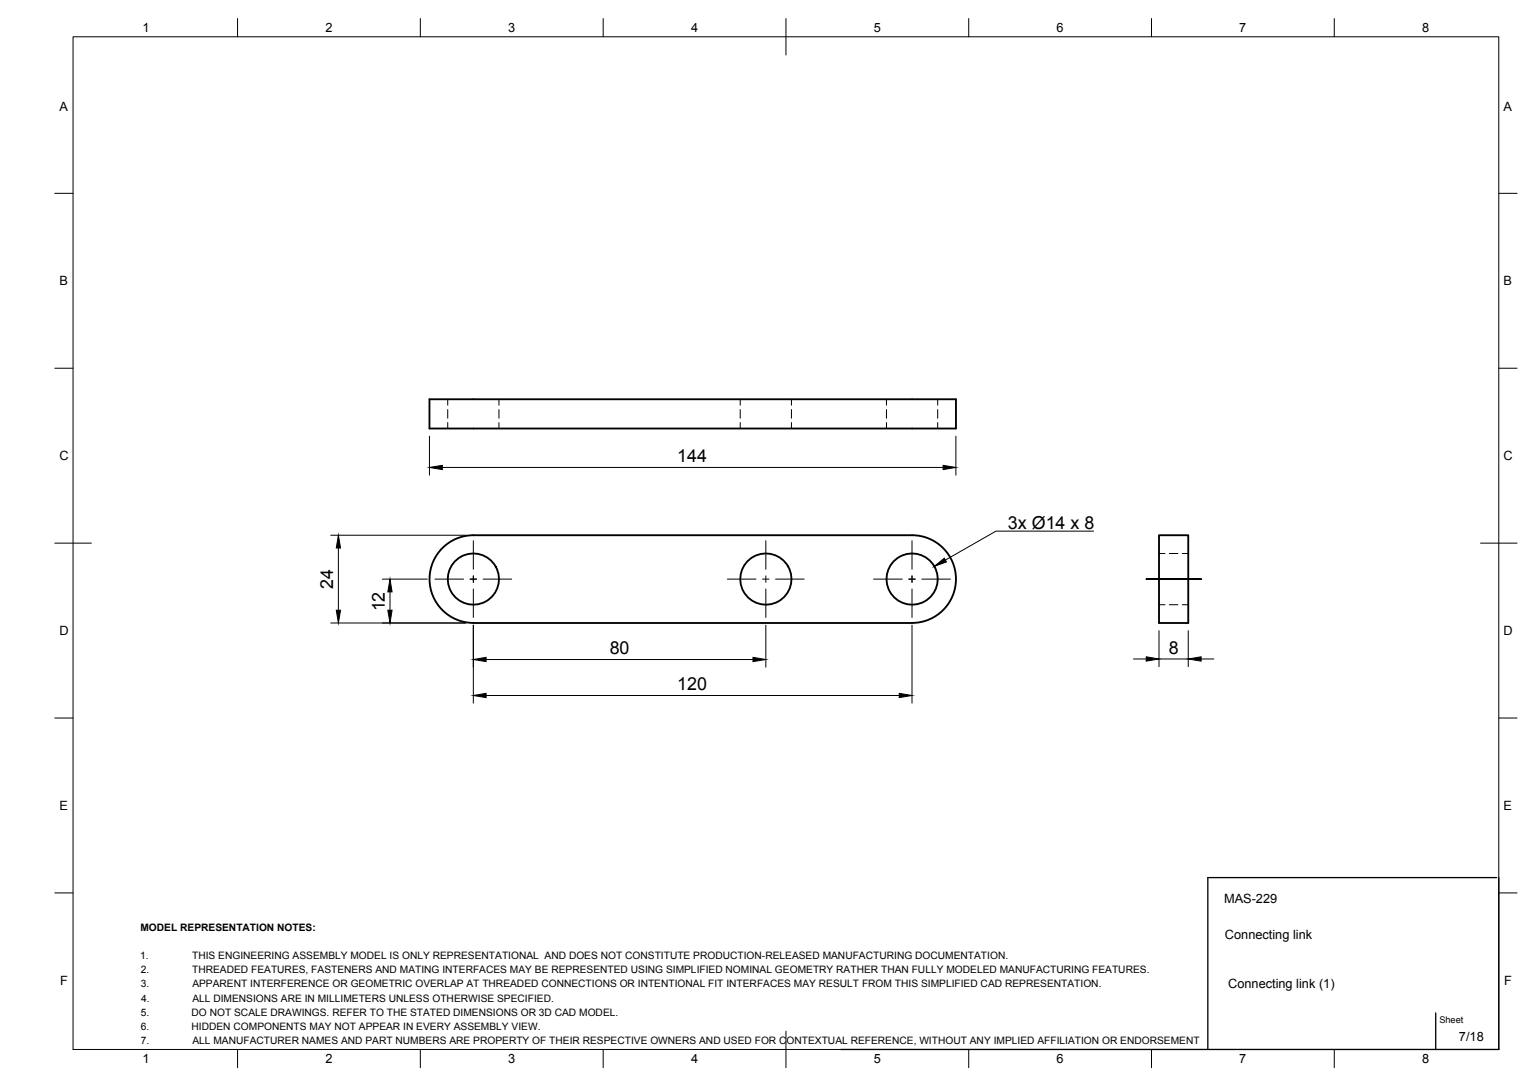
ISO-10303-21;
HEADER;
/* Generated by software containing ST-Developer
 * from STEP Tools, Inc. (www.steptools.com) 
 */

FILE_DESCRIPTION(
/* description */ ('Independently dimensioned six-bar single-leg walking-linkage demonstr
ator. Whole-mm20 crank,60 upper rocker,80/120 ternary coupler,120 lowe
r rocker,140 knee pitch and260 toe reach; ground pivots0/0,60/0,40/60.
 Seven native revolutes close both loops. Four reused native library f
amilies, fully retained shared pins and layered real spacer stacks, bo
nded rubber toe. Benchtop reference mechanism; no complete vehicle, lo
ad, gait stability, adhesive, weld, fit or life rating.'),
/* implementation_level */ '2;1');

FILE_NAME(
/* name */ 'Connecting link.step',
/* time_stamp */ '2026-11-09T20:33:14-08:00',
/* author */ (''),
/* organization */ (''),
/* preprocessor_version */ 'ST-DEVELOPER v20.2',
/* originating_system */ 'Autodesk Translation Framework v15.17.0.0',
/* authorisation */ '');

FILE_SCHEMA (('AUTOMOTIVE_DESIGN { 1 0 10303 214 3 1 1 }'));
ENDSEC;

DATA;
#10=MECHANICAL_DESIGN_GEOMETRIC_PRESENTATION_REPRESENTATION('',(#259),#4048);
#223=SHAPE_REPRESENTATION_RELATIONSHIP('SRR','None',#4147,#241);
#241=ADVANCED_BREP_SHAPE_REPRESENTATION('',(#277),#4034);
#259=STYLED_ITEM('',(#4246),#277);
#277=MANIFOLD_SOLID_BREP('Body1',#2148);
#313=FACE_BOUND('',#608,.T.);
#314=FACE_BOUND('',#609,.T.);
#315=FACE_BOUND('',#610,.T.);
#316=FACE_BOUND('',#612,.T.);
#317=FACE_BOUND('',#613,.T.);
#318=FACE_BOUND('',#614,.T.);
#370=PLANE('',#2443);
#371=PLANE('',#2447);
#372=PLANE('',#2451);
#373=PLANE('',#2452);
#452=FACE_OUTER_BOUND('',#600,.T.);
#453=FACE_OUTER_BOUND('',#601,.T.);
#454=FACE_OUTER_BOUND('',#602,.T.);
#455=FACE_OUTER_BOUND('',#603,.T.);
#456=FACE_OUTER_BOUND('',#604,.T.);
#457=FACE_OUTER_BOUND('',#605,.T.);
#458=FACE_OUTER_BOUND('',#606,.T.);
#459=FACE_OUTER_BOUND('',#607,.T.);
#460=FACE_OUTER_BOUND('',#611,.T.);
#600=EDGE_LOOP('',(#1659,#1660,#1661,#1662));
#601=EDGE_LOOP('',(#1663,#1664,#1665,#1666));
#602=EDGE_LOOP('',(#1667,#1668,#1669,#1670));
#603=EDGE_LOOP('',(#1671,#1672,#1673,#1674));
#604=EDGE_LOOP('',(#1675,#1676,#1677,#1678));
#605=EDGE_LOOP('',(#1679,#1680,#1681,#1682));
#606=EDGE_LOOP('',(#1683,#1684,#1685,#1686));
#607=EDGE_LOOP('',(#1687,#1688,#1689,#1690));
#608=EDGE_LOOP('',(#1691));
#609=EDGE_LOOP('',(#1692));
#610=EDGE_LOOP('',(#1693));
#611=EDGE_LOOP('',(#1694,#1695,#1696,#1697));
#612=EDGE_LOOP('',(#1698));
#613=EDGE_LOOP('',(#1699));
#614=EDGE_LOOP('',(#1700));
#781=LINE('',#3608,#906);
#782=LINE('',#3614,#907);
#783=LINE('',#3620,#908);
#784=LINE('',#3625,#909);
#785=LINE('',#3627,#910);
#786=LINE('',#3629,#911);
#787=LINE('',#3630,#912);
#788=LINE('',#3636,#913);
#789=LINE('',#3639,#914);
#790=LINE('',#3641,#915);
#791=LINE('',#3642,#916);
#906=VECTOR('',#2878,7.);
#907=VECTOR('',#2885,7.);
#908=VECTOR('',#2892,7.);
#909=VECTOR('',#2897,10.);
#910=VECTOR('',#2898,10.);
#911=VECTOR('',#2899,10.);
#912=VECTOR('',#2900,10.);
#913=VECTOR('',#2907,10.);
#914=VECTOR('',#2910,10.);
#915=VECTOR('',#2911,10.);
#916=VECTOR('',#2912,10.);
#1004=CIRCLE('',#2435,7.);
#1005=CIRCLE('',#2436,7.);
#1006=CIRCLE('',#2438,7.);
#1007=CIRCLE('',#2439,7.);
#1008=CIRCLE('',#2441,7.);
#1009=CIRCLE('',#2442,7.);
#1010=CIRCLE('',#2445,12.);
#1011=CIRCLE('',#2446,12.);
#1012=CIRCLE('',#2449,12.);
#1013=CIRCLE('',#2450,12.);
#1146=VERTEX_POINT('',#3605);
#1147=VERTEX_POINT('',#3607);
#1148=VERTEX_POINT('',#3611);
#1149=VERTEX_POINT('',#3613);
#1150=VERTEX_POINT('',#3617);
#1151=VERTEX_POINT('',#3619);
#1152=VERTEX_POINT('',#3623);
#1153=VERTEX_POINT('',#3624);
#1154=VERTEX_POINT('',#3626);
#1155=VERTEX_POINT('',#3628);
#1156=VERTEX_POINT('',#3632);
#1157=VERTEX_POINT('',#3634);
#1158=VERTEX_POINT('',#3638);
#1159=VERTEX_POINT('',#3640);
#1333=EDGE_CURVE('',#1146,#1146,#1004,.T.);
#1334=EDGE_CURVE('',#1146,#1147,#781,.T.);
#1335=EDGE_CURVE('',#1147,#1147,#1005,.T.);
#1336=EDGE_CURVE('',#1148,#1148,#1006,.T.);
#1337=EDGE_CURVE('',#1148,#1149,#782,.T.);
#1338=EDGE_CURVE('',#1149,#1149,#1007,.T.);
#1339=EDGE_CURVE('',#1150,#1150,#1008,.T.);
#1340=EDGE_CURVE('',#1150,#1151,#783,.T.);
#1341=EDGE_CURVE('',#1151,#1151,#1009,.T.);
#1342=EDGE_CURVE('',#1152,#1153,#784,.T.);
#1343=EDGE_CURVE('',#1153,#1154,#785,.T.);
#1344=EDGE_CURVE('',#1155,#1154,#786,.T.);
#1345=EDGE_CURVE('',#1152,#1155,#787,.T.);
#1346=EDGE_CURVE('',#1156,#1152,#1010,.T.);
#1347=EDGE_CURVE('',#1157,#1155,#1011,.T.);
#1348=EDGE_CURVE('',#1156,#1157,#788,.T.);
#1349=EDGE_CURVE('',#1158,#1156,#789,.T.);
#1350=EDGE_CURVE('',#1159,#1157,#790,.T.);
#1351=EDGE_CURVE('',#1158,#1159,#791,.T.);
#1352=EDGE_CURVE('',#1153,#1158,#1012,.T.);
#1353=EDGE_CURVE('',#1154,#1159,#1013,.T.);
#1659=ORIENTED_EDGE('',*,*,#1333,.F.);
#1660=ORIENTED_EDGE('',*,*,#1334,.T.);
#1661=ORIENTED_EDGE('',*,*,#1335,.F.);
#1662=ORIENTED_EDGE('',*,*,#1334,.F.);
#1663=ORIENTED_EDGE('',*,*,#1336,.F.);
#1664=ORIENTED_EDGE('',*,*,#1337,.T.);
#1665=ORIENTED_EDGE('',*,*,#1338,.F.);
#1666=ORIENTED_EDGE('',*,*,#1337,.F.);
#1667=ORIENTED_EDGE('',*,*,#1339,.F.);
#1668=ORIENTED_EDGE('',*,*,#1340,.T.);
#1669=ORIENTED_EDGE('',*,*,#1341,.F.);
#1670=ORIENTED_EDGE('',*,*,#1340,.F.);
#1671=ORIENTED_EDGE('',*,*,#1342,.T.);
#1672=ORIENTED_EDGE('',*,*,#1343,.T.);
#1673=ORIENTED_EDGE('',*,*,#1344,.F.);
#1674=ORIENTED_EDGE('',*,*,#1345,.F.);
#1675=ORIENTED_EDGE('',*,*,#1346,.T.);
#1676=ORIENTED_EDGE('',*,*,#1345,.T.);
#1677=ORIENTED_EDGE('',*,*,#1347,.F.);
#1678=ORIENTED_EDGE('',*,*,#1348,.F.);
#1679=ORIENTED_EDGE('',*,*,#1349,.T.);
#1680=ORIENTED_EDGE('',*,*,#1348,.T.);
#1681=ORIENTED_EDGE('',*,*,#1350,.F.);
#1682=ORIENTED_EDGE('',*,*,#1351,.F.);
#1683=ORIENTED_EDGE('',*,*,#1352,.T.);
#1684=ORIENTED_EDGE('',*,*,#1351,.T.);
#1685=ORIENTED_EDGE('',*,*,#1353,.F.);
#1686=ORIENTED_EDGE('',*,*,#1343,.F.);
#1687=ORIENTED_EDGE('',*,*,#1353,.T.);
#1688=ORIENTED_EDGE('',*,*,#1350,.T.);
#1689=ORIENTED_EDGE('',*,*,#1347,.T.);
#1690=ORIENTED_EDGE('',*,*,#1344,.T.);
#1691=ORIENTED_EDGE('',*,*,#1333,.T.);
#1692=ORIENTED_EDGE('',*,*,#1336,.T.);
#1693=ORIENTED_EDGE('',*,*,#1339,.T.);
#1694=ORIENTED_EDGE('',*,*,#1352,.F.);
#1695=ORIENTED_EDGE('',*,*,#1342,.F.);
#1696=ORIENTED_EDGE('',*,*,#1346,.F.);
#1697=ORIENTED_EDGE('',*,*,#1349,.F.);
#1698=ORIENTED_EDGE('',*,*,#1335,.T.);
#1699=ORIENTED_EDGE('',*,*,#1338,.T.);
#1700=ORIENTED_EDGE('',*,*,#1341,.T.);
#1978=CYLINDRICAL_SURFACE('',#2434,7.);
#1979=CYLINDRICAL_SURFACE('',#2437,7.);
#1980=CYLINDRICAL_SURFACE('',#2440,7.);
#1981=CYLINDRICAL_SURFACE('',#2444,12.);
#1982=CYLINDRICAL_SURFACE('',#2448,12.);
#2055=ADVANCED_FACE('',(#452),#1978,.F.);
#2056=ADVANCED_FACE('',(#453),#1979,.F.);
#2057=ADVANCED_FACE('',(#454),#1980,.F.);
#2058=ADVANCED_FACE('',(#455),#370,.T.);
#2059=ADVANCED_FACE('',(#456),#1981,.T.);
#2060=ADVANCED_FACE('',(#457),#371,.T.);
#2061=ADVANCED_FACE('',(#458),#1982,.T.);
#2062=ADVANCED_FACE('',(#459,#313,#314,#315),#372,.T.);
#2063=ADVANCED_FACE('',(#460,#316,#317,#318),#373,.F.);
#2148=CLOSED_SHELL('',(#2055,#2056,#2057,#2058,#2059,#2060,#2061,#2062,
#2063));
#2433=AXIS2_PLACEMENT_3D('',#3603,#2872,#2873);
#2434=AXIS2_PLACEMENT_3D('',#3604,#2874,#2875);
#2435=AXIS2_PLACEMENT_3D('',#3606,#2876,#2877);
#2436=AXIS2_PLACEMENT_3D('',#3609,#2879,#2880);
#2437=AXIS2_PLACEMENT_3D('',#3610,#2881,#2882);
#2438=AXIS2_PLACEMENT_3D('',#3612,#2883,#2884);
#2439=AXIS2_PLACEMENT_3D('',#3615,#2886,#2887);
#2440=AXIS2_PLACEMENT_3D('',#3616,#2888,#2889);
#2441=AXIS2_PLACEMENT_3D('',#3618,#2890,#2891);
#2442=AXIS2_PLACEMENT_3D('',#3621,#2893,#2894);
#2443=AXIS2_PLACEMENT_3D('',#3622,#2895,#2896);
#2444=AXIS2_PLACEMENT_3D('',#3631,#2901,#2902);
#2445=AXIS2_PLACEMENT_3D('',#3633,#2903,#2904);
#2446=AXIS2_PLACEMENT_3D('',#3635,#2905,#2906);
#2447=AXIS2_PLACEMENT_3D('',#3637,#2908,#2909);
#2448=AXIS2_PLACEMENT_3D('',#3643,#2913,#2914);
#2449=AXIS2_PLACEMENT_3D('',#3644,#2915,#2916);
#2450=AXIS2_PLACEMENT_3D('',#3645,#2917,#2918);
#2451=AXIS2_PLACEMENT_3D('',#3646,#2919,#2920);
#2452=AXIS2_PLACEMENT_3D('',#3647,#2921,#2922);
#2872=DIRECTION('axis',(0.,0.,1.));
#2873=DIRECTION('refdir',(1.,0.,0.));
#2874=DIRECTION('center_axis',(0.,0.,-1.));
#2875=DIRECTION('ref_axis',(1.,0.,0.));
#2876=DIRECTION('center_axis',(0.,0.,-1.));
#2877=DIRECTION('ref_axis',(1.,0.,0.));
#2878=DIRECTION('',(0.,0.,-1.));
#2879=DIRECTION('center_axis',(0.,0.,1.));
#2880=DIRECTION('ref_axis',(1.,0.,0.));
#2881=DIRECTION('center_axis',(0.,0.,-1.));
#2882=DIRECTION('ref_axis',(1.,0.,0.));
#2883=DIRECTION('center_axis',(0.,0.,-1.));
#2884=DIRECTION('ref_axis',(1.,0.,0.));
#2885=DIRECTION('',(0.,0.,-1.));
#2886=DIRECTION('center_axis',(0.,0.,1.));
#2887=DIRECTION('ref_axis',(1.,0.,0.));
#2888=DIRECTION('center_axis',(0.,0.,-1.));
#2889=DIRECTION('ref_axis',(1.,0.,0.));
#2890=DIRECTION('center_axis',(0.,0.,-1.));
#2891=DIRECTION('ref_axis',(1.,0.,0.));
#2892=DIRECTION('',(0.,0.,-1.));
#2893=DIRECTION('center_axis',(0.,0.,1.));
#2894=DIRECTION('ref_axis',(1.,0.,0.));
#2895=DIRECTION('center_axis',(0.,1.,0.));
#2896=DIRECTION('ref_axis',(-1.,0.,0.));
#2897=DIRECTION('',(-1.,0.,0.));
#2898=DIRECTION('',(0.,0.,1.));
#2899=DIRECTION('',(-1.,0.,0.));
#2900=DIRECTION('',(0.,0.,1.));
#2901=DIRECTION('center_axis',(0.,0.,1.));
#2902=DIRECTION('ref_axis',(0.,-1.,0.));
#2903=DIRECTION('center_axis',(0.,0.,1.));
#2904=DIRECTION('ref_axis',(0.,-1.,0.));
#2905=DIRECTION('center_axis',(0.,0.,1.));
#2906=DIRECTION('ref_axis',(0.,-1.,0.));
#2907=DIRECTION('',(0.,0.,1.));
#2908=DIRECTION('center_axis',(0.,-1.,0.));
#2909=DIRECTION('ref_axis',(1.,0.,0.));
#2910=DIRECTION('',(1.,0.,0.));
#2911=DIRECTION('',(1.,0.,0.));
#2912=DIRECTION('',(0.,0.,1.));
#2913=DIRECTION('center_axis',(0.,0.,1.));
#2914=DIRECTION('ref_axis',(0.,1.,0.));
#2915=DIRECTION('center_axis',(0.,0.,1.));
#2916=DIRECTION('ref_axis',(0.,1.,0.));
#2917=DIRECTION('center_axis',(0.,0.,1.));
#2918=DIRECTION('ref_axis',(0.,1.,0.));
#2919=DIRECTION('center_axis',(0.,0.,1.));
#2920=DIRECTION('ref_axis',(1.,0.,0.));
#2921=DIRECTION('center_axis',(0.,0.,1.));
#2922=DIRECTION('ref_axis',(1.,0.,0.));
#3603=CARTESIAN_POINT('',(0.,0.,0.));
#3604=CARTESIAN_POINT('Origin',(80.,0.,4.));
#3605=CARTESIAN_POINT('',(73.,8.57252759403147E-16,8.));
#3606=CARTESIAN_POINT('Origin',(80.,0.,8.));
#3607=CARTESIAN_POINT('',(73.,8.57252759403147E-16,0.));
#3608=CARTESIAN_POINT('',(73.,8.57252759403147E-16,4.));
#3609=CARTESIAN_POINT('Origin',(80.,0.,0.));
#3610=CARTESIAN_POINT('Origin',(0.,0.,4.));
#3611=CARTESIAN_POINT('',(-7.,8.57252759403147E-16,8.));
#3612=CARTESIAN_POINT('Origin',(0.,0.,8.));
#3613=CARTESIAN_POINT('',(-7.,8.57252759403147E-16,0.));
#3614=CARTESIAN_POINT('',(-7.,8.57252759403147E-16,4.));
#3615=CARTESIAN_POINT('Origin',(0.,0.,0.));
#3616=CARTESIAN_POINT('Origin',(120.,0.,4.));
#3617=CARTESIAN_POINT('',(113.,8.57252759403147E-16,8.));
#3618=CARTESIAN_POINT('Origin',(120.,0.,8.));
#3619=CARTESIAN_POINT('',(113.,8.57252759403147E-16,0.));
#3620=CARTESIAN_POINT('',(113.,8.57252759403147E-16,4.));
#3621=CARTESIAN_POINT('Origin',(120.,0.,0.));
#3622=CARTESIAN_POINT('Origin',(120.,12.,0.));
#3623=CARTESIAN_POINT('',(120.,12.,0.));
#3624=CARTESIAN_POINT('',(0.,12.,0.));
#3625=CARTESIAN_POINT('',(120.,12.,0.));
#3626=CARTESIAN_POINT('',(0.,12.,8.));
#3627=CARTESIAN_POINT('',(0.,12.,0.));
#3628=CARTESIAN_POINT('',(120.,12.,8.));
#3629=CARTESIAN_POINT('',(120.,12.,8.));
#3630=CARTESIAN_POINT('',(120.,12.,0.));
#3631=CARTESIAN_POINT('Origin',(120.,-1.11022302462516E-15,0.));
#3632=CARTESIAN_POINT('',(120.,-12.,0.));
#3633=CARTESIAN_POINT('Origin',(120.,-1.11022302462516E-15,0.));
#3634=CARTESIAN_POINT('',(120.,-12.,8.));
#3635=CARTESIAN_POINT('Origin',(120.,-1.11022302462516E-15,8.));
#3636=CARTESIAN_POINT('',(120.,-12.,0.));
#3637=CARTESIAN_POINT('Origin',(0.,-12.,0.));
#3638=CARTESIAN_POINT('',(-1.46957615897682E-15,-12.,0.));
#3639=CARTESIAN_POINT('',(0.,-12.,0.));
#3640=CARTESIAN_POINT('',(-1.46957615897682E-15,-12.,8.));
#3641=CARTESIAN_POINT('',(0.,-12.,8.));
#3642=CARTESIAN_POINT('',(-1.46957615897682E-15,-12.,0.));
#3643=CARTESIAN_POINT('Origin',(0.,0.,0.));
#3644=CARTESIAN_POINT('Origin',(0.,0.,0.));
#3645=CARTESIAN_POINT('Origin',(0.,0.,8.));
#3646=CARTESIAN_POINT('Origin',(60.,0.,8.));
#3647=CARTESIAN_POINT('Origin',(60.,0.,0.));
#4014=UNCERTAINTY_MEASURE_WITH_UNIT(LENGTH_MEASURE(0.01),#4049,
'DISTANCE_ACCURACY_VALUE',
'Maximum model space distance between geometric entities at asserted c
onnectivities');
#4028=UNCERTAINTY_MEASURE_WITH_UNIT(LENGTH_MEASURE(0.01),#4049,
'DISTANCE_ACCURACY_VALUE',
'Maximum model space distance between geometric entities at asserted c
onnectivities');
#4034=(
GEOMETRIC_REPRESENTATION_CONTEXT(3)
GLOBAL_UNCERTAINTY_ASSIGNED_CONTEXT((#4014))
GLOBAL_UNIT_ASSIGNED_CONTEXT((#4049,#4051,#4052))
REPRESENTATION_CONTEXT('','3D')
);
#4048=(
GEOMETRIC_REPRESENTATION_CONTEXT(3)
GLOBAL_UNCERTAINTY_ASSIGNED_CONTEXT((#4028))
GLOBAL_UNIT_ASSIGNED_CONTEXT((#4049,#4051,#4052))
REPRESENTATION_CONTEXT('','3D')
);
#4049=(
LENGTH_UNIT()
NAMED_UNIT(*)
SI_UNIT(.MILLI.,.METRE.)
);
#4051=(
NAMED_UNIT(*)
PLANE_ANGLE_UNIT()
SI_UNIT($,.RADIAN.)
);
#4052=(
NAMED_UNIT(*)
SI_UNIT($,.STERADIAN.)
SOLID_ANGLE_UNIT()
);
#4058=SHAPE_DEFINITION_REPRESENTATION(#4077,#4147);
#4077=PRODUCT_DEFINITION_SHAPE('',$,#4167);
#4147=SHAPE_REPRESENTATION('',(#2433),#4034);
#4161=PRODUCT_DEFINITION_CONTEXT('part definition',#4220,'design');
#4167=PRODUCT_DEFINITION('Connecting link','Connecting link',#4186,#4161);
#4186=PRODUCT_DEFINITION_FORMATION('',$,#4227);
#4220=APPLICATION_CONTEXT(
'Core Data for Automotive Mechanical Design Process');
#4221=PRODUCT_CONTEXT('part definition',#4220,'mechanical');
#4227=PRODUCT('Connecting link','Connecting link','Connecting link',(#4221));
#4246=PRESENTATION_STYLE_ASSIGNMENT((#4260));
#4260=SURFACE_STYLE_USAGE(.BOTH.,#4274);
#4274=SURFACE_SIDE_STYLE('',(#4288));
#4288=SURFACE_STYLE_FILL_AREA(#4302);
#4302=FILL_AREA_STYLE('Connecting link finish',(#4316));
#4316=FILL_AREA_STYLE_COLOUR('Connecting link finish',#4330);
#4330=COLOUR_RGB('Connecting link finish',0.662745098039216,0.831372549019608,
0.949019607843137);
ENDSEC;
END-ISO-10303-21;
